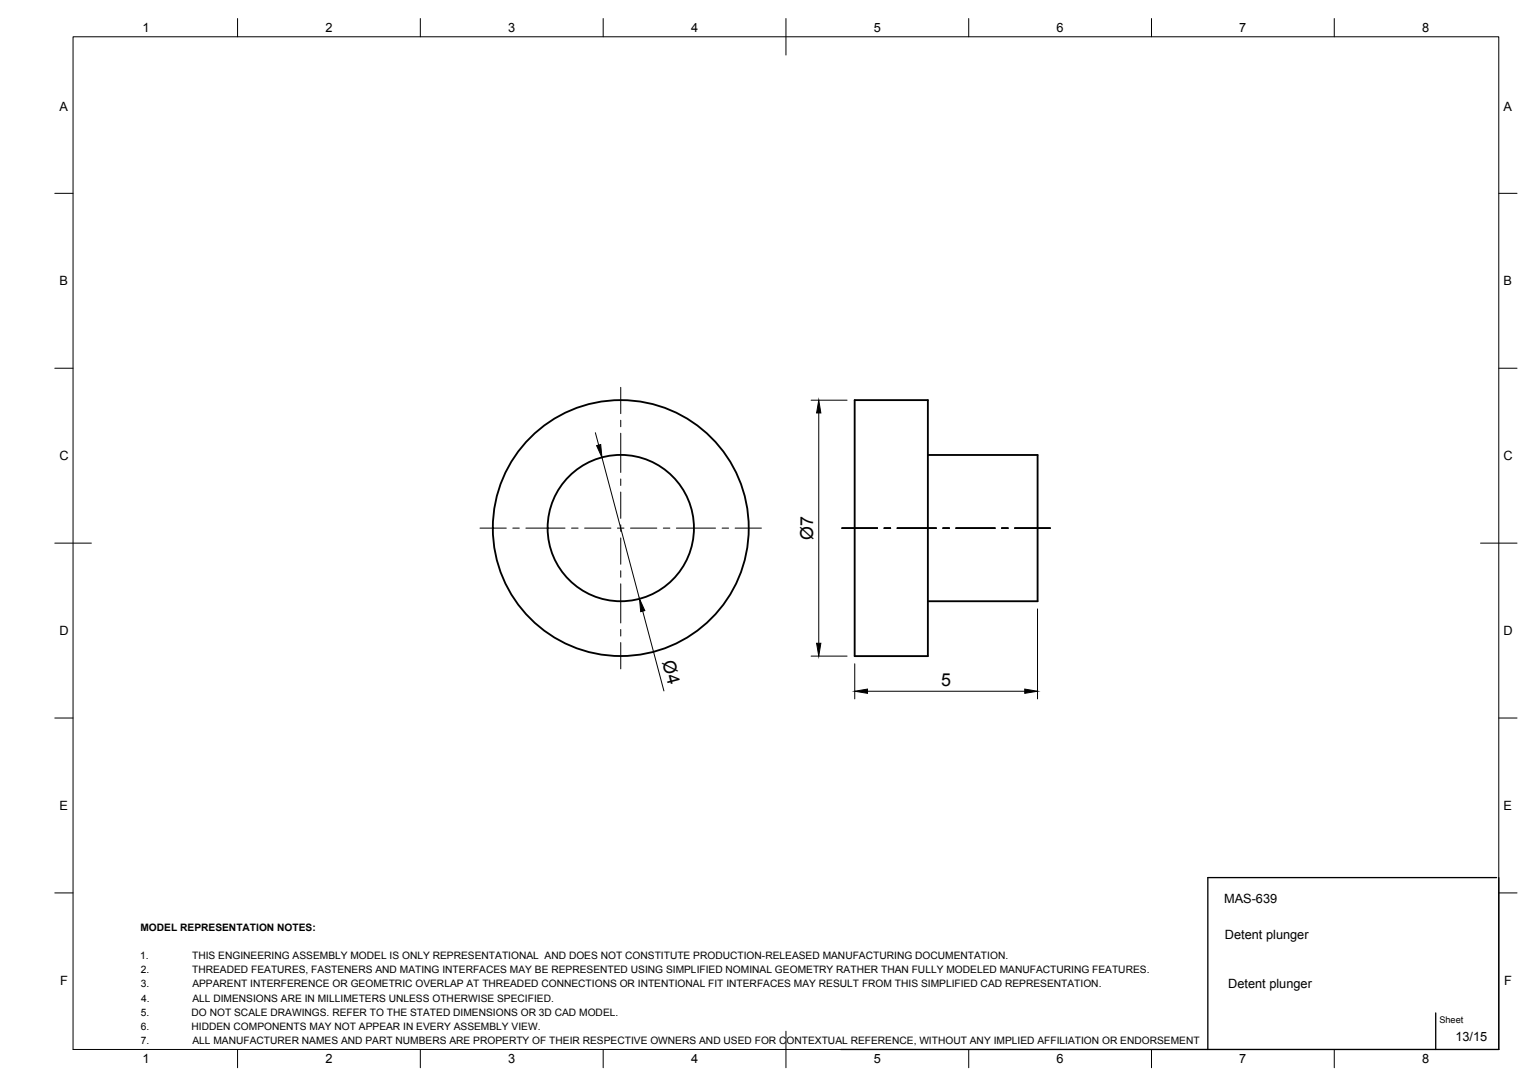
ISO-10303-21;
HEADER;
/* Generated by software containing ST-Developer
 * from STEP Tools, Inc. (www.steptools.com) 
 */

FILE_DESCRIPTION(
/* description */ ('Independent maintained push-to-latch/pull-to-reset mushroom-operator 
CAD. Two opposed spring-loaded ball detents in turned circular seats b
ias both travel stops; direct normally-closed bridge opens6mm when pre
ssed. Rounded palm/pull rim, captured head screw, removable detent clo
sures, native Coil spring families, insulated shared terminals and ord
inary machining features. Manual geometric states and ideal same-mater
ial spring-energy direction only; no electrical/safety certification, 
force/contact dynamics, wear, load or life rating. Requested blue/gray
 visual palette, not safety identification. External wiring/anchors an
d application engineering omitted.'),
/* implementation_level */ '2;1');

FILE_NAME(
/* name */ 'Detent plunger.step',
/* time_stamp */ '2026-11-08T17:54:26-08:00',
/* author */ (''),
/* organization */ (''),
/* preprocessor_version */ 'ST-DEVELOPER v20.2',
/* originating_system */ 'Autodesk Translation Framework v15.17.0.0',
/* authorisation */ '');

FILE_SCHEMA (('AUTOMOTIVE_DESIGN { 1 0 10303 214 3 1 1 }'));
ENDSEC;

DATA;
#10=MECHANICAL_DESIGN_GEOMETRIC_PRESENTATION_REPRESENTATION('',(#201),#43980);
#167=SHAPE_REPRESENTATION_RELATIONSHIP('SRR','None',#44067,#184);
#184=ADVANCED_BREP_SHAPE_REPRESENTATION('',(#218),#43974);
#201=STYLED_ITEM('',(#44159),#218);
#218=MANIFOLD_SOLID_BREP('Body1',#11242);
#322=FACE_BOUND('',#1629,.T.);
#439=PLANE('',#12039);
#440=PLANE('',#12044);
#441=PLANE('',#12047);
#942=FACE_OUTER_BOUND('',#1628,.T.);
#943=FACE_OUTER_BOUND('',#1630,.T.);
#944=FACE_OUTER_BOUND('',#1631,.T.);
#945=FACE_OUTER_BOUND('',#1632,.T.);
#946=FACE_OUTER_BOUND('',#1633,.T.);
#1628=EDGE_LOOP('',(#9325));
#1629=EDGE_LOOP('',(#9326));
#1630=EDGE_LOOP('',(#9327,#9328,#9329,#9330));
#1631=EDGE_LOOP('',(#9331));
#1632=EDGE_LOOP('',(#9332,#9333,#9334,#9335));
#1633=EDGE_LOOP('',(#9336));
#1958=CIRCLE('',#12040,0.35);
#1959=CIRCLE('',#12041,0.2);
#1960=CIRCLE('',#12043,0.35);
#1961=CIRCLE('',#12046,0.2);
#3288=LINE('',#35905,#3920);
#3289=LINE('',#35909,#3921);
#3920=VECTOR('',#13941,0.35);
#3921=VECTOR('',#13946,0.2);
#4914=VERTEX_POINT('',#35898);
#4915=VERTEX_POINT('',#35900);
#4916=VERTEX_POINT('',#35903);
#4917=VERTEX_POINT('',#35908);
#6432=EDGE_CURVE('',#4914,#4914,#1958,.T.);
#6433=EDGE_CURVE('',#4915,#4915,#1959,.T.);
#6434=EDGE_CURVE('',#4916,#4916,#1960,.T.);
#6435=EDGE_CURVE('',#4916,#4914,#3288,.T.);
#6436=EDGE_CURVE('',#4915,#4917,#3289,.T.);
#6437=EDGE_CURVE('',#4917,#4917,#1961,.T.);
#9325=ORIENTED_EDGE('',*,*,#6432,.F.);
#9326=ORIENTED_EDGE('',*,*,#6433,.T.);
#9327=ORIENTED_EDGE('',*,*,#6434,.F.);
#9328=ORIENTED_EDGE('',*,*,#6435,.T.);
#9329=ORIENTED_EDGE('',*,*,#6432,.T.);
#9330=ORIENTED_EDGE('',*,*,#6435,.F.);
#9331=ORIENTED_EDGE('',*,*,#6434,.T.);
#9332=ORIENTED_EDGE('',*,*,#6433,.F.);
#9333=ORIENTED_EDGE('',*,*,#6436,.T.);
#9334=ORIENTED_EDGE('',*,*,#6437,.T.);
#9335=ORIENTED_EDGE('',*,*,#6436,.F.);
#9336=ORIENTED_EDGE('',*,*,#6437,.F.);
#10503=CYLINDRICAL_SURFACE('',#12042,0.35);
#10504=CYLINDRICAL_SURFACE('',#12045,0.2);
#11067=ADVANCED_FACE('',(#942,#322),#439,.F.);
#11068=ADVANCED_FACE('',(#943),#10503,.T.);
#11069=ADVANCED_FACE('',(#944),#440,.T.);
#11070=ADVANCED_FACE('',(#945),#10504,.T.);
#11071=ADVANCED_FACE('',(#946),#441,.F.);
#11242=CLOSED_SHELL('',(#11067,#11068,#11069,#11070,#11071));
#12038=AXIS2_PLACEMENT_3D('',#35896,#13929,#13930);
#12039=AXIS2_PLACEMENT_3D('',#35897,#13931,#13932);
#12040=AXIS2_PLACEMENT_3D('',#35899,#13933,#13934);
#12041=AXIS2_PLACEMENT_3D('',#35901,#13935,#13936);
#12042=AXIS2_PLACEMENT_3D('',#35902,#13937,#13938);
#12043=AXIS2_PLACEMENT_3D('',#35904,#13939,#13940);
#12044=AXIS2_PLACEMENT_3D('',#35906,#13942,#13943);
#12045=AXIS2_PLACEMENT_3D('',#35907,#13944,#13945);
#12046=AXIS2_PLACEMENT_3D('',#35910,#13947,#13948);
#12047=AXIS2_PLACEMENT_3D('',#35911,#13949,#13950);
#13929=DIRECTION('axis',(0.,0.,1.));
#13930=DIRECTION('refdir',(1.,0.,0.));
#13931=DIRECTION('center_axis',(0.,0.,1.));
#13932=DIRECTION('ref_axis',(1.,0.,0.));
#13933=DIRECTION('center_axis',(0.,0.,1.));
#13934=DIRECTION('ref_axis',(1.,0.,0.));
#13935=DIRECTION('center_axis',(0.,0.,1.));
#13936=DIRECTION('ref_axis',(1.,0.,0.));
#13937=DIRECTION('center_axis',(0.,0.,1.));
#13938=DIRECTION('ref_axis',(1.,0.,0.));
#13939=DIRECTION('center_axis',(0.,0.,1.));
#13940=DIRECTION('ref_axis',(1.,0.,0.));
#13941=DIRECTION('',(0.,0.,-1.));
#13942=DIRECTION('center_axis',(0.,0.,1.));
#13943=DIRECTION('ref_axis',(1.,0.,0.));
#13944=DIRECTION('center_axis',(0.,0.,1.));
#13945=DIRECTION('ref_axis',(1.,0.,0.));
#13946=DIRECTION('',(0.,0.,-1.));
#13947=DIRECTION('center_axis',(0.,0.,1.));
#13948=DIRECTION('ref_axis',(1.,0.,0.));
#13949=DIRECTION('center_axis',(0.,0.,1.));
#13950=DIRECTION('ref_axis',(1.,0.,0.));
#35896=CARTESIAN_POINT('',(0.,0.,0.));
#35897=CARTESIAN_POINT('Origin',(0.,0.,0.3));
#35898=CARTESIAN_POINT('',(-0.35,-4.28626379701574E-17,0.3));
#35899=CARTESIAN_POINT('Origin',(0.,0.,0.3));
#35900=CARTESIAN_POINT('',(-0.2,-2.44929359829471E-17,0.3));
#35901=CARTESIAN_POINT('Origin',(0.,0.,0.3));
#35902=CARTESIAN_POINT('Origin',(0.,0.,0.3));
#35903=CARTESIAN_POINT('',(-0.35,-4.28626379701574E-17,0.5));
#35904=CARTESIAN_POINT('Origin',(0.,0.,0.5));
#35905=CARTESIAN_POINT('',(-0.35,-4.28626379701574E-17,0.3));
#35906=CARTESIAN_POINT('Origin',(0.,0.,0.5));
#35907=CARTESIAN_POINT('Origin',(0.,0.,0.));
#35908=CARTESIAN_POINT('',(-0.2,-2.44929359829471E-17,0.));
#35909=CARTESIAN_POINT('',(-0.2,-2.44929359829471E-17,0.));
#35910=CARTESIAN_POINT('Origin',(0.,0.,0.));
#35911=CARTESIAN_POINT('Origin',(0.,0.,0.));
#43955=UNCERTAINTY_MEASURE_WITH_UNIT(LENGTH_MEASURE(0.001),#43981,
'DISTANCE_ACCURACY_VALUE',
'Maximum model space distance between geometric entities at asserted c
onnectivities');
#43961=UNCERTAINTY_MEASURE_WITH_UNIT(LENGTH_MEASURE(0.001),#43981,
'DISTANCE_ACCURACY_VALUE',
'Maximum model space distance between geometric entities at asserted c
onnectivities');
#43974=(
GEOMETRIC_REPRESENTATION_CONTEXT(3)
GLOBAL_UNCERTAINTY_ASSIGNED_CONTEXT((#43955))
GLOBAL_UNIT_ASSIGNED_CONTEXT((#43981,#43983,#43984))
REPRESENTATION_CONTEXT('','3D')
);
#43980=(
GEOMETRIC_REPRESENTATION_CONTEXT(3)
GLOBAL_UNCERTAINTY_ASSIGNED_CONTEXT((#43961))
GLOBAL_UNIT_ASSIGNED_CONTEXT((#43981,#43983,#43984))
REPRESENTATION_CONTEXT('','3D')
);
#43981=(
LENGTH_UNIT()
NAMED_UNIT(*)
SI_UNIT(.CENTI.,.METRE.)
);
#43983=(
NAMED_UNIT(*)
PLANE_ANGLE_UNIT()
SI_UNIT($,.RADIAN.)
);
#43984=(
NAMED_UNIT(*)
SI_UNIT($,.STERADIAN.)
SOLID_ANGLE_UNIT()
);
#43997=SHAPE_DEFINITION_REPRESENTATION(#44015,#44067);
#44015=PRODUCT_DEFINITION_SHAPE('',$,#44086);
#44067=SHAPE_REPRESENTATION('',(#12038),#43974);
#44073=PRODUCT_DEFINITION_CONTEXT('part definition',#44129,'design');
#44086=PRODUCT_DEFINITION('Detent plunger','Detent plunger',#44104,#44073);
#44104=PRODUCT_DEFINITION_FORMATION('',$,#44143);
#44129=APPLICATION_CONTEXT(
'Core Data for Automotive Mechanical Design Process');
#44130=PRODUCT_CONTEXT('part definition',#44129,'mechanical');
#44143=PRODUCT('Detent plunger','Detent plunger',$,(#44130));
#44159=PRESENTATION_STYLE_ASSIGNMENT((#44171));
#44171=SURFACE_STYLE_USAGE(.BOTH.,#44183);
#44183=SURFACE_SIDE_STYLE('',(#44195));
#44195=SURFACE_STYLE_FILL_AREA(#44207);
#44207=FILL_AREA_STYLE('Plunger gray',(#44219));
#44219=FILL_AREA_STYLE_COLOUR('Plunger gray',#44231);
#44231=COLOUR_RGB('Plunger gray',0.576470588235294,0.615686274509804,0.666666666666667);
ENDSEC;
END-ISO-10303-21;
